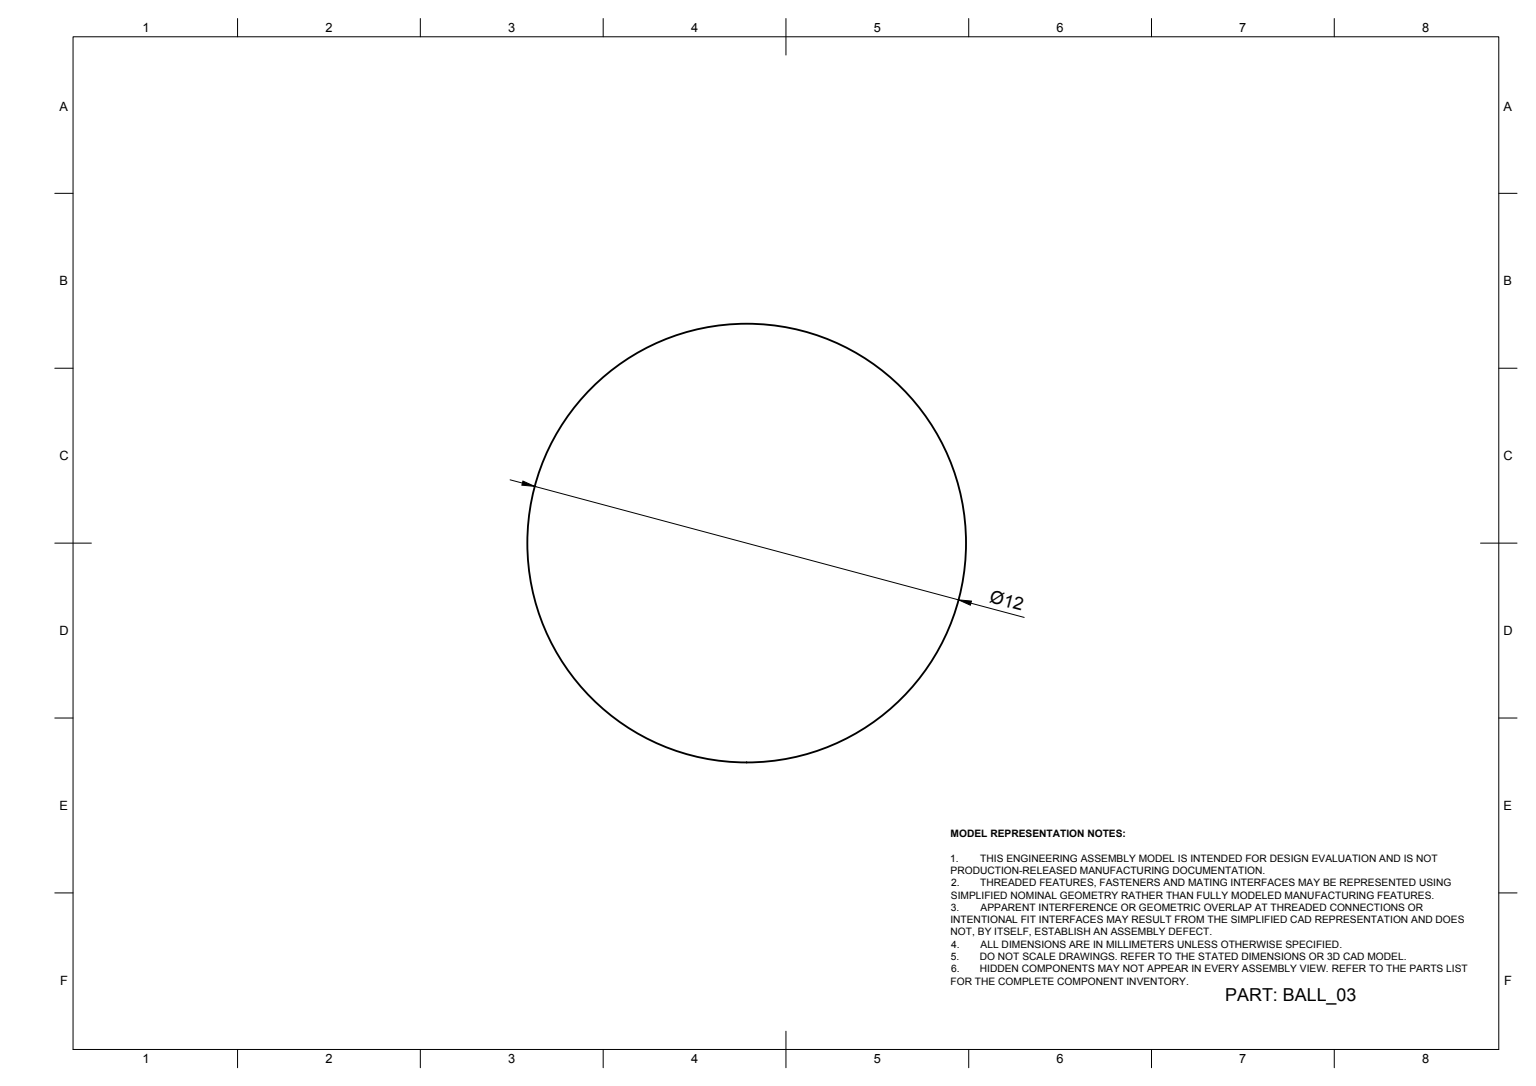
ISO-10303-21;
HEADER;
/* Generated by software containing ST-Developer
 * from STEP Tools, Inc. (www.steptools.com) 
 */

FILE_DESCRIPTION(
/* description */ (''),
/* implementation_level */ '2;1');

FILE_NAME(
/* name */ 'Ball_03.step',
/* time_stamp */ '2026-10-05T00:14:20-07:00',
/* author */ (''),
/* organization */ (''),
/* preprocessor_version */ 'ST-DEVELOPER v20.2',
/* originating_system */ 'Autodesk Translation Framework v15.15.0.0',
/* authorisation */ '');

FILE_SCHEMA (('AUTOMOTIVE_DESIGN { 1 0 10303 214 3 1 1 }'));
ENDSEC;

DATA;
#10=MECHANICAL_DESIGN_GEOMETRIC_PRESENTATION_REPRESENTATION('',(#3374),#75336);
#3354=SPHERICAL_SURFACE('',#32141,6.);
#3358=SHAPE_REPRESENTATION_RELATIONSHIP('SRR','None',#75371,#3366);
#3366=ADVANCED_BREP_SHAPE_REPRESENTATION('',(#3382),#75331);
#3374=STYLED_ITEM('',(#75418),#3382);
#3382=MANIFOLD_SOLID_BREP('Body1',#32024);
#3404=CIRCLE('',#32142,6.);
#5148=FACE_OUTER_BOUND('',#6876,.T.);
#6876=EDGE_LOOP('',(#19629,#19630));
#11112=VERTEX_POINT('',#46110);
#11113=VERTEX_POINT('',#46111);
#14509=EDGE_CURVE('',#11112,#11113,#3404,.T.);
#19629=ORIENTED_EDGE('',*,*,#14509,.T.);
#19630=ORIENTED_EDGE('',*,*,#14509,.F.);
#30308=ADVANCED_FACE('',(#5148),#3354,.T.);
#32024=CLOSED_SHELL('',(#30308));
#32140=AXIS2_PLACEMENT_3D('',#46108,#36411,#36412);
#32141=AXIS2_PLACEMENT_3D('',#46109,#36413,#36414);
#32142=AXIS2_PLACEMENT_3D('',#46112,#36415,#36416);
#36411=DIRECTION('axis',(0.,0.,1.));
#36412=DIRECTION('refdir',(1.,0.,0.));
#36413=DIRECTION('center_axis',(0.,0.,1.));
#36414=DIRECTION('ref_axis',(-0.5,-0.866025403784438,0.));
#36415=DIRECTION('center_axis',(-0.866025403784439,0.5,0.));
#36416=DIRECTION('ref_axis',(0.5,0.866025403784439,0.));
#46108=CARTESIAN_POINT('',(0.,0.,0.));
#46109=CARTESIAN_POINT('Origin',(-15.,-25.9807621135331,13.));
#46110=CARTESIAN_POINT('',(-15.,-25.9807621135331,19.));
#46111=CARTESIAN_POINT('',(-15.,-25.9807621135331,6.99999999999999));
#46112=CARTESIAN_POINT('Origin',(-15.,-25.9807621135331,13.));
#75321=UNCERTAINTY_MEASURE_WITH_UNIT(LENGTH_MEASURE(0.01),#75337,
'DISTANCE_ACCURACY_VALUE',
'Maximum model space distance between geometric entities at asserted c
onnectivities');
#75326=UNCERTAINTY_MEASURE_WITH_UNIT(LENGTH_MEASURE(0.01),#75337,
'DISTANCE_ACCURACY_VALUE',
'Maximum model space distance between geometric entities at asserted c
onnectivities');
#75331=(
GEOMETRIC_REPRESENTATION_CONTEXT(3)
GLOBAL_UNCERTAINTY_ASSIGNED_CONTEXT((#75321))
GLOBAL_UNIT_ASSIGNED_CONTEXT((#75337,#75339,#75340))
REPRESENTATION_CONTEXT('','3D')
);
#75336=(
GEOMETRIC_REPRESENTATION_CONTEXT(3)
GLOBAL_UNCERTAINTY_ASSIGNED_CONTEXT((#75326))
GLOBAL_UNIT_ASSIGNED_CONTEXT((#75337,#75339,#75340))
REPRESENTATION_CONTEXT('','3D')
);
#75337=(
LENGTH_UNIT()
NAMED_UNIT(*)
SI_UNIT(.MILLI.,.METRE.)
);
#75339=(
NAMED_UNIT(*)
PLANE_ANGLE_UNIT()
SI_UNIT($,.RADIAN.)
);
#75340=(
NAMED_UNIT(*)
SI_UNIT($,.STERADIAN.)
SOLID_ANGLE_UNIT()
);
#75345=SHAPE_DEFINITION_REPRESENTATION(#75354,#75371);
#75354=PRODUCT_DEFINITION_SHAPE('',$,#75381);
#75371=SHAPE_REPRESENTATION('',(#32140),#75331);
#75376=PRODUCT_DEFINITION_CONTEXT('part definition',#75405,'design');
#75381=PRODUCT_DEFINITION('Ball_03','Ball_03',#75390,#75376);
#75390=PRODUCT_DEFINITION_FORMATION('',$,#75411);
#75405=APPLICATION_CONTEXT(
'Core Data for Automotive Mechanical Design Process');
#75406=PRODUCT_CONTEXT('part definition',#75405,'mechanical');
#75411=PRODUCT('Ball_03','Ball_03',$,(#75406));
#75418=PRESENTATION_STYLE_ASSIGNMENT((#75422));
#75422=SURFACE_STYLE_USAGE(.BOTH.,#75426);
#75426=SURFACE_SIDE_STYLE('',(#75430));
#75430=SURFACE_STYLE_FILL_AREA(#75434);
#75434=FILL_AREA_STYLE('Opaque(200,203,41)',(#75438));
#75438=FILL_AREA_STYLE_COLOUR('Opaque(200,203,41)',#75442);
#75442=COLOUR_RGB('Opaque(200,203,41)', 0.66274510, 0.83137255, 0.94901961);
ENDSEC;
END-ISO-10303-21;
